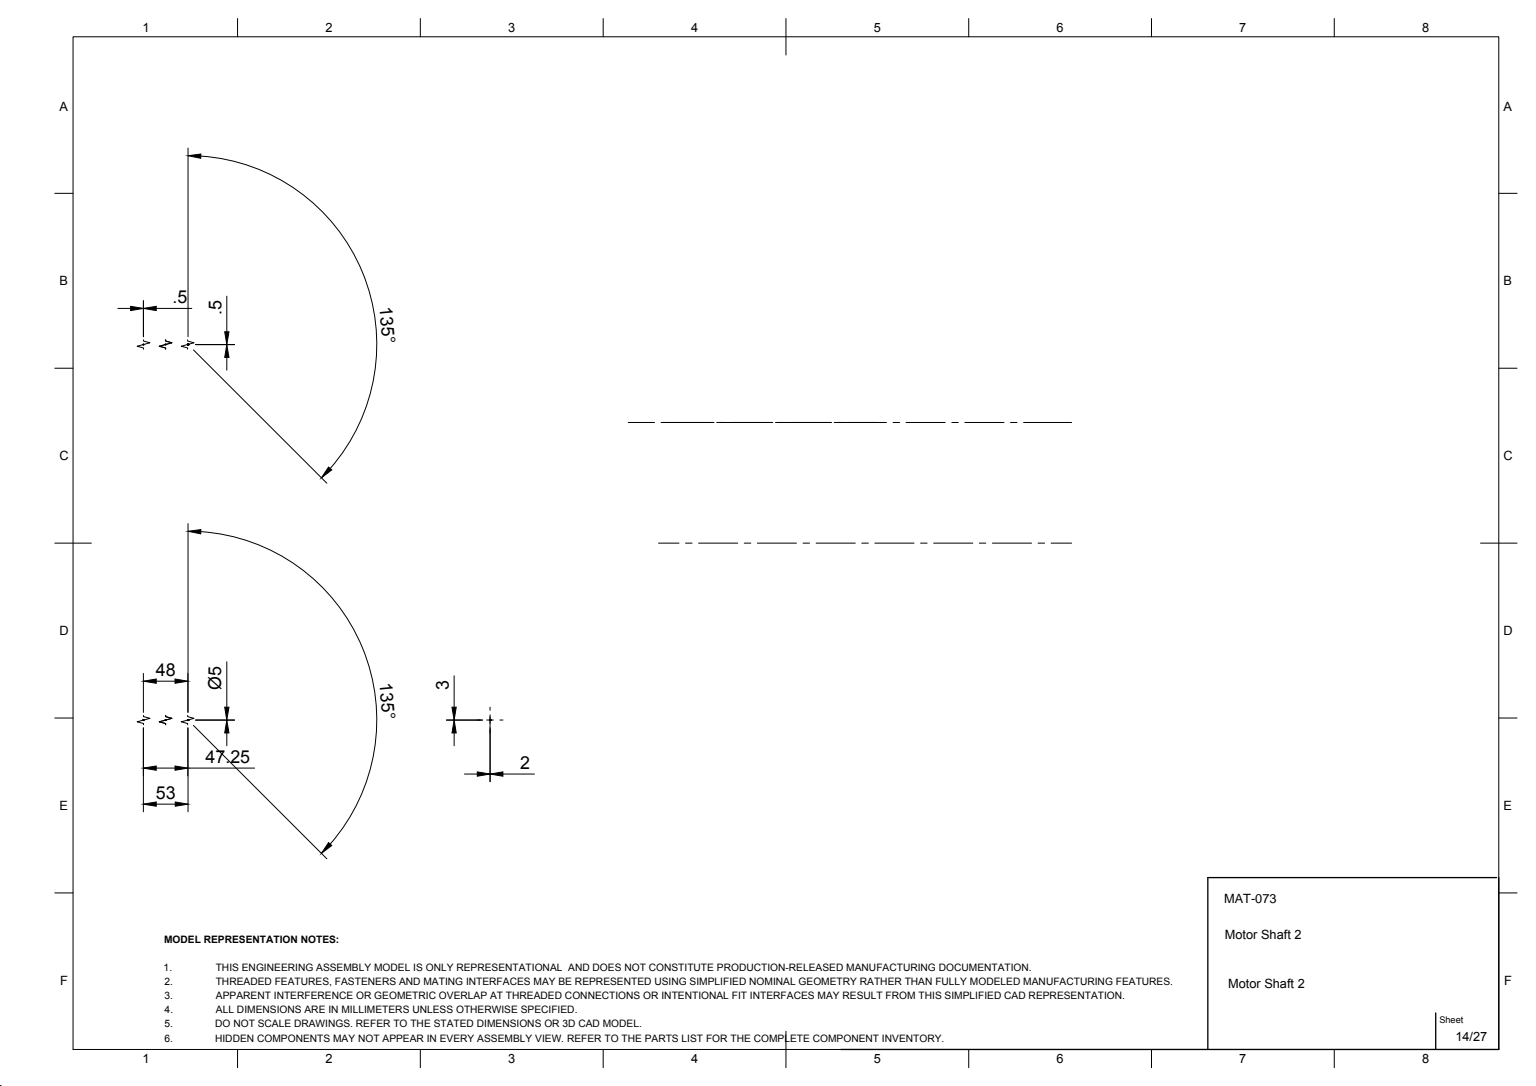
ISO-10303-21;
HEADER;
/* Generated by software containing ST-Developer
 * from STEP Tools, Inc. (www.steptools.com) 
 */

FILE_DESCRIPTION(
/* description */ ('CAx-IF Rec.Pracs.---Representation and Presentation of Product Manufa
cturing Information (PMI)---4.0---2014-10-13'),
/* implementation_level */ '2;1');

FILE_NAME(
/* name */ 'Motor Shaft 2.step',
/* time_stamp */ '2026-10-24T18:52:33-07:00',
/* author */ (''),
/* organization */ (''),
/* preprocessor_version */ 'ST-DEVELOPER v20.2',
/* originating_system */ 'Autodesk Translation Framework v15.17.0.0',
/* authorisation */ '');

FILE_SCHEMA (('AP242_MANAGED_MODEL_BASED_3D_ENGINEERING_MIM_LF { 1 0 10303 442 2 1 4 }'));
ENDSEC;

DATA;
#10=MECHANICAL_DESIGN_GEOMETRIC_PRESENTATION_REPRESENTATION('',(#427),#34876);
#156=(
BOUNDED_CURVE()
B_SPLINE_CURVE(2,(#31813,#31814,#31815),.UNSPECIFIED.,.F.,.F.)
B_SPLINE_CURVE_WITH_KNOTS((3,3),(0.,0.159611859165466),.UNSPECIFIED.)
CURVE()
GEOMETRIC_REPRESENTATION_ITEM()
RATIONAL_B_SPLINE_CURVE((1.,1.06066017177976,1.))
REPRESENTATION_ITEM('')
);
#157=(
BOUNDED_CURVE()
B_SPLINE_CURVE(2,(#31820,#31821,#31822),.UNSPECIFIED.,.F.,.F.)
B_SPLINE_CURVE_WITH_KNOTS((3,3),(0.159611859165466,0.319223718330933),
 .UNSPECIFIED.)
CURVE()
GEOMETRIC_REPRESENTATION_ITEM()
RATIONAL_B_SPLINE_CURVE((1.,1.06066017177976,1.))
REPRESENTATION_ITEM('')
);
#185=CONICAL_SURFACE('',#21171,0.00225,0.78539816339745);
#186=CONICAL_SURFACE('',#21175,0.00225,0.78539816339745);
#187=CONICAL_SURFACE('',#21192,0.00225,0.78539816339745);
#361=SHAPE_REPRESENTATION_RELATIONSHIP('SRR','None',#34998,#394);
#394=ADVANCED_BREP_SHAPE_REPRESENTATION('',(#460),#34856);
#427=STYLED_ITEM('',(#35159),#460);
#460=MANIFOLD_SOLID_BREP('Motor Shaft 2',#19567);
#534=FACE_BOUND('',#6448,.T.);
#535=FACE_BOUND('',#6450,.T.);
#861=PLANE('',#21181);
#862=PLANE('',#21183);
#863=PLANE('',#21187);
#864=PLANE('',#21188);
#865=PLANE('',#21194);
#866=PLANE('',#21195);
#1899=LINE('',#31807,#3498);
#1900=LINE('',#31828,#3499);
#1901=LINE('',#31838,#3500);
#1902=LINE('',#31839,#3501);
#1903=LINE('',#31841,#3502);
#1904=LINE('',#31844,#3503);
#1905=LINE('',#31848,#3504);
#1906=LINE('',#31854,#3505);
#3498=VECTOR('',#25516,0.00225);
#3499=VECTOR('',#25533,0.002);
#3500=VECTOR('',#25546,1.);
#3501=VECTOR('',#25547,0.0025);
#3502=VECTOR('',#25548,1.);
#3503=VECTOR('',#25553,1.);
#3504=VECTOR('',#25558,0.0025);
#3505=VECTOR('',#25565,0.00225);
#4547=CYLINDRICAL_SURFACE('',#21178,0.002);
#4548=CYLINDRICAL_SURFACE('',#21185,0.0025);
#4549=CYLINDRICAL_SURFACE('',#21189,0.0025);
#5345=FACE_OUTER_BOUND('',#6444,.T.);
#5346=FACE_OUTER_BOUND('',#6445,.T.);
#5347=FACE_OUTER_BOUND('',#6446,.T.);
#5348=FACE_OUTER_BOUND('',#6447,.T.);
#5349=FACE_OUTER_BOUND('',#6449,.T.);
#5350=FACE_OUTER_BOUND('',#6451,.T.);
#5351=FACE_OUTER_BOUND('',#6452,.T.);
#5352=FACE_OUTER_BOUND('',#6453,.T.);
#5353=FACE_OUTER_BOUND('',#6454,.T.);
#5354=FACE_OUTER_BOUND('',#6455,.T.);
#5355=FACE_OUTER_BOUND('',#6456,.T.);
#5356=FACE_OUTER_BOUND('',#6457,.T.);
#6444=EDGE_LOOP('',(#15784,#15785,#15786,#15787,#15788));
#6445=EDGE_LOOP('',(#15789,#15790,#15791,#15792));
#6446=EDGE_LOOP('',(#15793,#15794,#15795,#15796));
#6447=EDGE_LOOP('',(#15797));
#6448=EDGE_LOOP('',(#15798));
#6449=EDGE_LOOP('',(#15799));
#6450=EDGE_LOOP('',(#15800));
#6451=EDGE_LOOP('',(#15801,#15802,#15803,#15804,#15805,#15806,#15807,#15808,
#15809));
#6452=EDGE_LOOP('',(#15810,#15811,#15812,#15813,#15814));
#6453=EDGE_LOOP('',(#15815,#15816));
#6454=EDGE_LOOP('',(#15817,#15818,#15819,#15820,#15821));
#6455=EDGE_LOOP('',(#15822,#15823,#15824,#15825,#15826));
#6456=EDGE_LOOP('',(#15827));
#6457=EDGE_LOOP('',(#15828,#15829));
#7534=CIRCLE('',#21172,0.00250000000001);
#7535=CIRCLE('',#21173,0.00250000000001);
#7536=CIRCLE('',#21174,0.00200000000001);
#7537=CIRCLE('',#21176,0.00200000000001);
#7538=CIRCLE('',#21177,0.00250000000001);
#7539=CIRCLE('',#21179,0.00200000000001);
#7540=CIRCLE('',#21180,0.00200000000001);
#7541=CIRCLE('',#21182,0.00250000000001);
#7542=CIRCLE('',#21184,0.00250000000001);
#7543=CIRCLE('',#21186,0.00250000000001);
#7544=CIRCLE('',#21190,0.00250000000001);
#7545=CIRCLE('',#21191,0.00250000000001);
#7546=CIRCLE('',#21193,0.00200000000001);
#9058=VERTEX_POINT('',#31805);
#9059=VERTEX_POINT('',#31806);
#9060=VERTEX_POINT('',#31808);
#9061=VERTEX_POINT('',#31810);
#9062=VERTEX_POINT('',#31812);
#9063=VERTEX_POINT('',#31819);
#9064=VERTEX_POINT('',#31825);
#9065=VERTEX_POINT('',#31827);
#9066=VERTEX_POINT('',#31831);
#9067=VERTEX_POINT('',#31834);
#9068=VERTEX_POINT('',#31837);
#9069=VERTEX_POINT('',#31840);
#9070=VERTEX_POINT('',#31847);
#9071=VERTEX_POINT('',#31849);
#9072=VERTEX_POINT('',#31853);
#11450=EDGE_CURVE('',#9058,#9059,#1899,.T.);
#11451=EDGE_CURVE('',#9058,#9060,#7534,.T.);
#11452=EDGE_CURVE('',#9060,#9061,#7535,.T.);
#11453=EDGE_CURVE('',#9061,#9062,#156,.T.);
#11454=EDGE_CURVE('',#9062,#9059,#7536,.T.);
#11455=EDGE_CURVE('',#9059,#9062,#7537,.T.);
#11456=EDGE_CURVE('',#9062,#9063,#157,.T.);
#11457=EDGE_CURVE('',#9063,#9058,#7538,.T.);
#11458=EDGE_CURVE('',#9064,#9064,#7539,.T.);
#11459=EDGE_CURVE('',#9064,#9065,#1900,.T.);
#11460=EDGE_CURVE('',#9065,#9065,#7540,.T.);
#11461=EDGE_CURVE('',#9066,#9066,#7541,.T.);
#11462=EDGE_CURVE('',#9067,#9067,#7542,.T.);
#11463=EDGE_CURVE('',#9068,#9061,#1901,.T.);
#11464=EDGE_CURVE('',#9060,#9067,#1902,.T.);
#11465=EDGE_CURVE('',#9063,#9069,#1903,.T.);
#11466=EDGE_CURVE('',#9069,#9068,#7543,.T.);
#11467=EDGE_CURVE('',#9068,#9069,#1904,.T.);
#11468=EDGE_CURVE('',#9066,#9070,#1905,.T.);
#11469=EDGE_CURVE('',#9071,#9070,#7544,.T.);
#11470=EDGE_CURVE('',#9070,#9071,#7545,.T.);
#11471=EDGE_CURVE('',#9071,#9072,#1906,.T.);
#11472=EDGE_CURVE('',#9072,#9072,#7546,.T.);
#15784=ORIENTED_EDGE('',*,*,#11450,.F.);
#15785=ORIENTED_EDGE('',*,*,#11451,.T.);
#15786=ORIENTED_EDGE('',*,*,#11452,.T.);
#15787=ORIENTED_EDGE('',*,*,#11453,.T.);
#15788=ORIENTED_EDGE('',*,*,#11454,.T.);
#15789=ORIENTED_EDGE('',*,*,#11450,.T.);
#15790=ORIENTED_EDGE('',*,*,#11455,.T.);
#15791=ORIENTED_EDGE('',*,*,#11456,.T.);
#15792=ORIENTED_EDGE('',*,*,#11457,.T.);
#15793=ORIENTED_EDGE('',*,*,#11458,.T.);
#15794=ORIENTED_EDGE('',*,*,#11459,.T.);
#15795=ORIENTED_EDGE('',*,*,#11460,.T.);
#15796=ORIENTED_EDGE('',*,*,#11459,.F.);
#15797=ORIENTED_EDGE('',*,*,#11461,.F.);
#15798=ORIENTED_EDGE('',*,*,#11460,.F.);
#15799=ORIENTED_EDGE('',*,*,#11462,.F.);
#15800=ORIENTED_EDGE('',*,*,#11458,.F.);
#15801=ORIENTED_EDGE('',*,*,#11463,.T.);
#15802=ORIENTED_EDGE('',*,*,#11452,.F.);
#15803=ORIENTED_EDGE('',*,*,#11464,.T.);
#15804=ORIENTED_EDGE('',*,*,#11462,.T.);
#15805=ORIENTED_EDGE('',*,*,#11464,.F.);
#15806=ORIENTED_EDGE('',*,*,#11451,.F.);
#15807=ORIENTED_EDGE('',*,*,#11457,.F.);
#15808=ORIENTED_EDGE('',*,*,#11465,.T.);
#15809=ORIENTED_EDGE('',*,*,#11466,.T.);
#15810=ORIENTED_EDGE('',*,*,#11453,.F.);
#15811=ORIENTED_EDGE('',*,*,#11463,.F.);
#15812=ORIENTED_EDGE('',*,*,#11467,.T.);
#15813=ORIENTED_EDGE('',*,*,#11465,.F.);
#15814=ORIENTED_EDGE('',*,*,#11456,.F.);
#15815=ORIENTED_EDGE('',*,*,#11466,.F.);
#15816=ORIENTED_EDGE('',*,*,#11467,.F.);
#15817=ORIENTED_EDGE('',*,*,#11461,.T.);
#15818=ORIENTED_EDGE('',*,*,#11468,.T.);
#15819=ORIENTED_EDGE('',*,*,#11469,.F.);
#15820=ORIENTED_EDGE('',*,*,#11470,.F.);
#15821=ORIENTED_EDGE('',*,*,#11468,.F.);
#15822=ORIENTED_EDGE('',*,*,#11470,.T.);
#15823=ORIENTED_EDGE('',*,*,#11471,.T.);
#15824=ORIENTED_EDGE('',*,*,#11472,.T.);
#15825=ORIENTED_EDGE('',*,*,#11471,.F.);
#15826=ORIENTED_EDGE('',*,*,#11469,.T.);
#15827=ORIENTED_EDGE('',*,*,#11472,.F.);
#15828=ORIENTED_EDGE('',*,*,#11454,.F.);
#15829=ORIENTED_EDGE('',*,*,#11455,.F.);
#19061=ADVANCED_FACE('',(#5345),#185,.T.);
#19062=ADVANCED_FACE('',(#5346),#186,.T.);
#19063=ADVANCED_FACE('',(#5347),#4547,.T.);
#19064=ADVANCED_FACE('',(#5348,#534),#861,.F.);
#19065=ADVANCED_FACE('',(#5349,#535),#862,.T.);
#19066=ADVANCED_FACE('',(#5350),#4548,.T.);
#19067=ADVANCED_FACE('',(#5351),#863,.F.);
#19068=ADVANCED_FACE('',(#5352),#864,.F.);
#19069=ADVANCED_FACE('',(#5353),#4549,.T.);
#19070=ADVANCED_FACE('',(#5354),#187,.T.);
#19071=ADVANCED_FACE('',(#5355),#865,.F.);
#19072=ADVANCED_FACE('',(#5356),#866,.T.);
#19567=CLOSED_SHELL('',(#19061,#19062,#19063,#19064,#19065,#19066,#19067,
#19068,#19069,#19070,#19071,#19072));
#21170=AXIS2_PLACEMENT_3D('',#31803,#25512,#25513);
#21171=AXIS2_PLACEMENT_3D('',#31804,#25514,#25515);
#21172=AXIS2_PLACEMENT_3D('',#31809,#25517,#25518);
#21173=AXIS2_PLACEMENT_3D('',#31811,#25519,#25520);
#21174=AXIS2_PLACEMENT_3D('',#31816,#25521,#25522);
#21175=AXIS2_PLACEMENT_3D('',#31817,#25523,#25524);
#21176=AXIS2_PLACEMENT_3D('',#31818,#25525,#25526);
#21177=AXIS2_PLACEMENT_3D('',#31823,#25527,#25528);
#21178=AXIS2_PLACEMENT_3D('',#31824,#25529,#25530);
#21179=AXIS2_PLACEMENT_3D('',#31826,#25531,#25532);
#21180=AXIS2_PLACEMENT_3D('',#31829,#25534,#25535);
#21181=AXIS2_PLACEMENT_3D('',#31830,#25536,#25537);
#21182=AXIS2_PLACEMENT_3D('',#31832,#25538,#25539);
#21183=AXIS2_PLACEMENT_3D('',#31833,#25540,#25541);
#21184=AXIS2_PLACEMENT_3D('',#31835,#25542,#25543);
#21185=AXIS2_PLACEMENT_3D('',#31836,#25544,#25545);
#21186=AXIS2_PLACEMENT_3D('',#31842,#25549,#25550);
#21187=AXIS2_PLACEMENT_3D('',#31843,#25551,#25552);
#21188=AXIS2_PLACEMENT_3D('',#31845,#25554,#25555);
#21189=AXIS2_PLACEMENT_3D('',#31846,#25556,#25557);
#21190=AXIS2_PLACEMENT_3D('',#31850,#25559,#25560);
#21191=AXIS2_PLACEMENT_3D('',#31851,#25561,#25562);
#21192=AXIS2_PLACEMENT_3D('',#31852,#25563,#25564);
#21193=AXIS2_PLACEMENT_3D('',#31855,#25566,#25567);
#21194=AXIS2_PLACEMENT_3D('',#31856,#25568,#25569);
#21195=AXIS2_PLACEMENT_3D('',#31857,#25570,#25571);
#25512=DIRECTION('axis',(0.,0.,1.));
#25513=DIRECTION('refdir',(1.,0.,0.));
#25514=DIRECTION('center_axis',(6.65798752924967E-17,-1.,1.71022579061586E-31));
#25515=DIRECTION('ref_axis',(-0.211873077029416,-1.41064830464559E-17,0.97729719084324));
#25516=DIRECTION('',(-0.14981688951836,0.707106781186546,0.691053470879819));
#25517=DIRECTION('center_axis',(-6.65798752924967E-17,1.,-1.71022579061586E-31));
#25518=DIRECTION('ref_axis',(-0.211873077029416,-1.41064830464559E-17,0.977297190843239));
#25519=DIRECTION('center_axis',(-6.65798752924967E-17,1.,-1.71022579061586E-31));
#25520=DIRECTION('ref_axis',(-0.211873077029416,-1.41064830464559E-17,0.977297190843239));
#25521=DIRECTION('center_axis',(6.65798752924967E-17,-1.,1.71022579061586E-31));
#25522=DIRECTION('ref_axis',(-0.211873077029416,-1.41064830464559E-17,0.97729719084324));
#25523=DIRECTION('center_axis',(6.65798752924967E-17,-1.,1.71022579061586E-31));
#25524=DIRECTION('ref_axis',(-0.211873077029416,-1.41064830464559E-17,0.97729719084324));
#25525=DIRECTION('center_axis',(6.65798752924967E-17,-1.,1.71022579061586E-31));
#25526=DIRECTION('ref_axis',(-0.211873077029416,-1.41064830464559E-17,0.97729719084324));
#25527=DIRECTION('center_axis',(-6.65798752924967E-17,1.,-1.71022579061586E-31));
#25528=DIRECTION('ref_axis',(-0.211873077029416,-1.41064830464559E-17,0.977297190843239));
#25529=DIRECTION('center_axis',(-6.65798752924967E-17,1.,-1.71022579061586E-31));
#25530=DIRECTION('ref_axis',(0.211873077029416,1.41064830464559E-17,-0.977297190843239));
#25531=DIRECTION('center_axis',(6.65798752924967E-17,-1.,1.71022579061586E-31));
#25532=DIRECTION('ref_axis',(0.211873077029416,1.41064830464559E-17,-0.97729719084324));
#25533=DIRECTION('',(6.65798752924967E-17,-1.,1.71022579061586E-31));
#25534=DIRECTION('center_axis',(-6.65798752924967E-17,1.,-1.71022579061586E-31));
#25535=DIRECTION('ref_axis',(0.211873077029416,1.41064830464559E-17,-0.97729719084324));
#25536=DIRECTION('center_axis',(6.65798752924967E-17,-1.,1.71022579061586E-31));
#25537=DIRECTION('ref_axis',(0.97729719084324,6.50683250900503E-17,0.211873077029416));
#25538=DIRECTION('center_axis',(6.65798752924967E-17,-1.,1.71022579061586E-31));
#25539=DIRECTION('ref_axis',(0.211873077029416,1.41064830464559E-17,-0.977297190843239));
#25540=DIRECTION('center_axis',(6.65798752924967E-17,-1.,1.71022579061586E-31));
#25541=DIRECTION('ref_axis',(0.97729719084324,6.50683250900503E-17,0.211873077029416));
#25542=DIRECTION('center_axis',(-6.65798752924967E-17,1.,-1.71022579061586E-31));
#25543=DIRECTION('ref_axis',(0.211873077029416,1.41064830464559E-17,-0.977297190843239));
#25544=DIRECTION('center_axis',(-6.65798752924967E-17,1.,-1.71022579061586E-31));
#25545=DIRECTION('ref_axis',(0.211873077029416,1.41064830464559E-17,-0.97729719084324));
#25546=DIRECTION('',(-6.65798752924967E-17,1.,-1.71022579061586E-31));
#25547=DIRECTION('',(6.65798752924967E-17,-1.,1.71022579061586E-31));
#25548=DIRECTION('',(6.65798752924967E-17,-1.,1.71022579061586E-31));
#25549=DIRECTION('center_axis',(6.65798752924967E-17,-1.,1.71022579061586E-31));
#25550=DIRECTION('ref_axis',(0.211873077029416,1.41064830464559E-17,-0.977297190843239));
#25551=DIRECTION('center_axis',(-0.97729719084324,-6.50683250900503E-17,
-0.211873077029416));
#25552=DIRECTION('ref_axis',(-0.211873077029416,-1.06625068431886E-16,0.97729719084324));
#25553=DIRECTION('',(0.211873077028438,1.41064830463908E-17,-0.977297190843451));
#25554=DIRECTION('center_axis',(6.65798752924967E-17,-1.,1.71022579061586E-31));
#25555=DIRECTION('ref_axis',(0.97729719084324,6.50683250900503E-17,0.211873077029416));
#25556=DIRECTION('center_axis',(-6.65798752924967E-17,1.,-1.71022579061586E-31));
#25557=DIRECTION('ref_axis',(0.211873077029416,1.41064830464559E-17,-0.97729719084324));
#25558=DIRECTION('',(6.65798752924967E-17,-1.,1.71022579061586E-31));
#25559=DIRECTION('center_axis',(6.65798752924967E-17,-1.,1.71022579061586E-31));
#25560=DIRECTION('ref_axis',(-0.211873077029416,-1.41064830464559E-17,0.977297190843239));
#25561=DIRECTION('center_axis',(6.65798752924967E-17,-1.,1.71022579061586E-31));
#25562=DIRECTION('ref_axis',(-0.211873077029416,-1.41064830464559E-17,0.977297190843239));
#25563=DIRECTION('center_axis',(-6.65798752924967E-17,1.,-1.71022579061586E-31));
#25564=DIRECTION('ref_axis',(-0.211873077029416,-1.41064830464559E-17,0.97729719084324));
#25565=DIRECTION('',(-0.14981688951836,-0.707106781186546,0.691053470879819));
#25566=DIRECTION('center_axis',(-6.65798752924967E-17,1.,-1.71022579061586E-31));
#25567=DIRECTION('ref_axis',(-0.211873077029416,-1.41064830464559E-17,0.97729719084324));
#25568=DIRECTION('center_axis',(-6.65798752924967E-17,1.,-1.71022579061586E-31));
#25569=DIRECTION('ref_axis',(-0.211873077029416,-1.41064830464559E-17,0.97729719084324));
#25570=DIRECTION('center_axis',(-6.65798752924967E-17,1.,-1.71022579061586E-31));
#25571=DIRECTION('ref_axis',(-0.211873077029416,-1.41064830464559E-17,0.97729719084324));
#31803=CARTESIAN_POINT('',(0.,0.,0.));
#31804=CARTESIAN_POINT('Origin',(-4.68201057504096E-17,0.0215,5.80537005579265E-33));
#31805=CARTESIAN_POINT('',(0.000529682692573917,0.021249999999998,-0.00244324297711006));
#31806=CARTESIAN_POINT('',(0.000423746154058535,0.0217500000000012,-0.00195459438168533));
#31807=CARTESIAN_POINT('',(0.000476714423316139,0.0215,-0.00219891867939729));
#31808=CARTESIAN_POINT('',(-0.000529682692573586,0.02125000000001,0.0024432429771081));
#31809=CARTESIAN_POINT('Origin',(-4.68034607815872E-17,0.02125000000001,
5.84812570055634E-33));
#31810=CARTESIAN_POINT('',(0.00163678476614231,0.02125,0.00188969194032369));
#31811=CARTESIAN_POINT('Origin',(-4.68034607815872E-17,0.02125000000001,
5.84812570055634E-33));
#31812=CARTESIAN_POINT('',(0.00195459438168643,0.02175,0.000423746154058832));
#31813=CARTESIAN_POINT('Ctrl Pts',(0.00163678476614996,0.02125000000001,
0.00188969194033559));
#31814=CARTESIAN_POINT('Ctrl Pts',(0.00181334566367447,0.02175000000001,
0.0010752776146329));
#31815=CARTESIAN_POINT('Ctrl Pts',(0.00195459438169832,0.02175000000001,
0.000423746154051177));
#31816=CARTESIAN_POINT('Origin',(-4.68367507192334E-17,0.02175000000001,
5.76261441102555E-33));
#31817=CARTESIAN_POINT('Origin',(-4.68201057504096E-17,0.0215,5.80537005579265E-33));
#31818=CARTESIAN_POINT('Origin',(-4.68367507192334E-17,0.02175000000001,
5.76261441102555E-33));
#31819=CARTESIAN_POINT('',(0.00227240399723056,0.02125,-0.00104219963220603));
#31820=CARTESIAN_POINT('Ctrl Pts',(0.00195459438169832,0.02175000000001,
0.000423746154051177));
#31821=CARTESIAN_POINT('Ctrl Pts',(0.00209584309971794,0.02175000000001,
-0.000227785306511001));
#31822=CARTESIAN_POINT('Ctrl Pts',(0.00227240399724245,0.02125000000001,
-0.00104219963221369));
#31823=CARTESIAN_POINT('Origin',(-4.68034607815872E-17,0.02125000000001,
5.84812570055634E-33));
#31824=CARTESIAN_POINT('Origin',(-4.36409167051929E-17,-0.02625,1.39716982059834E-32));
#31825=CARTESIAN_POINT('',(-0.000423746154058875,-0.02550000000001,0.00195459438168648));
#31826=CARTESIAN_POINT('Origin',(-4.36908516116616E-17,-0.02550000000001,
1.38434312716889E-32));
#31827=CARTESIAN_POINT('',(-0.000423746154058875,-0.02625000000001,0.00195459438168648));
#31828=CARTESIAN_POINT('',(-0.000423746154058875,-0.02625,0.00195459438168648));
#31829=CARTESIAN_POINT('Origin',(-4.36409167051922E-17,-0.02625000000001,
1.39716982059851E-32));
#31830=CARTESIAN_POINT('Origin',(-4.36409167051929E-17,-0.02625,1.39716982059834E-32));
#31831=CARTESIAN_POINT('',(-0.000529682692573583,-0.02625000000001,0.0024432429771081));
#31832=CARTESIAN_POINT('Origin',(-4.36409167051922E-17,-0.02625000000001,
1.39716982059851E-32));
#31833=CARTESIAN_POINT('Origin',(-4.36908516116622E-17,-0.0255,1.38434312716872E-32));
#31834=CARTESIAN_POINT('',(-0.000529682692573583,-0.02550000000001,0.0024432429771081));
#31835=CARTESIAN_POINT('Origin',(-4.36908516116616E-17,-0.02550000000001,
1.38434312716889E-32));
#31836=CARTESIAN_POINT('Origin',(-4.50723840239816E-17,-0.00475,1.02947127561593E-32));
#31837=CARTESIAN_POINT('',(0.00163678476614231,0.00375,0.00188969194032369));
#31838=CARTESIAN_POINT('',(0.00163678476614996,-0.00475,0.00188969194033558));
#31839=CARTESIAN_POINT('',(-0.000529682692573585,-0.00475,0.0024432429771081));
#31840=CARTESIAN_POINT('',(0.00227240399723056,0.00375,-0.00104219963220603));
#31841=CARTESIAN_POINT('',(0.00227240399724245,-0.00475,-0.00104219963221368));
#31842=CARTESIAN_POINT('Origin',(-4.56383129639685E-17,0.00375000000001,
8.8410208341341E-33));
#31843=CARTESIAN_POINT('Origin',(0.00163678476614231,0.02175,0.00188969194032369));
#31844=CARTESIAN_POINT('',(0.00227240399724245,0.00375000000001,-0.00104219963221368));
#31845=CARTESIAN_POINT('Origin',(0.00219891867939725,0.00375,0.000476714423316185));
#31846=CARTESIAN_POINT('Origin',(-4.50723840239816E-17,-0.00475,1.02947127561593E-32));
#31847=CARTESIAN_POINT('',(-0.000529682692575702,-0.03075000000001,0.00244324297711787));
#31848=CARTESIAN_POINT('',(-0.000529682692573585,-0.00475,0.0024432429771081));
#31849=CARTESIAN_POINT('',(0.000529682692573497,-0.03075,-0.0024432429771081));
#31850=CARTESIAN_POINT('Origin',(-4.3341307266376E-17,-0.03075000000001,
1.47412998117623E-32));
#31851=CARTESIAN_POINT('Origin',(-4.3341307266376E-17,-0.03075000000001,
1.47412998117623E-32));
#31852=CARTESIAN_POINT('Origin',(-4.33246622975535E-17,-0.031,1.47840554565259E-32));
#31853=CARTESIAN_POINT('',(0.000423746154058788,-0.03125,-0.00195459438168648));
#31854=CARTESIAN_POINT('',(0.000476714423316142,-0.031,-0.00219891867939729));
#31855=CARTESIAN_POINT('Origin',(-4.33080173287297E-17,-0.03125000000001,
1.4826811101293E-32));
#31856=CARTESIAN_POINT('Origin',(-4.33080173287304E-17,-0.03125,1.48268111012913E-32));
#31857=CARTESIAN_POINT('Origin',(-4.68367507192327E-17,0.02175,5.76261441102726E-33));
#34821=UNCERTAINTY_MEASURE_WITH_UNIT(LENGTH_MEASURE(1.E-5),#34877,
'DISTANCE_ACCURACY_VALUE',
'Maximum model space distance between geometric entities at asserted c
onnectivities');
#34841=UNCERTAINTY_MEASURE_WITH_UNIT(LENGTH_MEASURE(1.E-5),#34877,
'DISTANCE_ACCURACY_VALUE',
'Maximum model space distance between geometric entities at asserted c
onnectivities');
#34856=(
GEOMETRIC_REPRESENTATION_CONTEXT(3)
GLOBAL_UNCERTAINTY_ASSIGNED_CONTEXT((#34821))
GLOBAL_UNIT_ASSIGNED_CONTEXT((#34877,#34878,#34879))
REPRESENTATION_CONTEXT('','3D')
);
#34876=(
GEOMETRIC_REPRESENTATION_CONTEXT(3)
GLOBAL_UNCERTAINTY_ASSIGNED_CONTEXT((#34841))
GLOBAL_UNIT_ASSIGNED_CONTEXT((#34877,#34878,#34879))
REPRESENTATION_CONTEXT('','3D')
);
#34877=(
LENGTH_UNIT()
NAMED_UNIT(*)
SI_UNIT($,.METRE.)
);
#34878=(
NAMED_UNIT(*)
PLANE_ANGLE_UNIT()
SI_UNIT($,.RADIAN.)
);
#34879=(
NAMED_UNIT(*)
SI_UNIT($,.STERADIAN.)
SOLID_ANGLE_UNIT()
);
#34894=SHAPE_DEFINITION_REPRESENTATION(#34928,#34998);
#34928=PRODUCT_DEFINITION_SHAPE('',$,#35033);
#34998=SHAPE_REPRESENTATION('',(#21170),#34856);
#35018=PRODUCT_DEFINITION_CONTEXT('part definition',#35122,'design');
#35033=PRODUCT_DEFINITION('Motor Shaft 2','Motor Shaft 2',#35067,#35018);
#35067=PRODUCT_DEFINITION_FORMATION('',$,#35138);
#35122=APPLICATION_CONTEXT('Managed model based 3d engineering');
#35123=PRODUCT_CONTEXT('part definition',#35122,'mechanical');
#35138=PRODUCT('Motor Shaft 2','Motor Shaft 2',
'LEGAL AND USAGE DISCLAIMER: this Data/Model is provided \X2\201C\X0\A
S IS\X2\201D\X0\ for informational and representational only. It is a 
geometric approximation and is NOT engineered, certified, or guarantee
d for dimensional accuracy, exact tolerances, or production-level prec
ision. Vendor disclaims all implied warranties including fitness for a
 particular purpose. DO NOT USE FOR DIRECT PHYSICAL MANUFACTURING, AUT
OMATED PRODUCTION, OR SAFETY-CRITICAL SYSTEMS without independent engi
neering verification and resolution of any design discrepancies.',(#35123));
#35159=PRESENTATION_STYLE_ASSIGNMENT((#35168));
#35168=SURFACE_STYLE_USAGE(.BOTH.,#35177);
#35177=SURFACE_SIDE_STYLE('',(#35186));
#35186=SURFACE_STYLE_FILL_AREA(#35195);
#35195=FILL_AREA_STYLE('Paint - Enamel Glossy (White)',(#35204));
#35204=FILL_AREA_STYLE_COLOUR('Paint - Enamel Glossy (White)',#35213);
#35213=COLOUR_RGB('Paint - Enamel Glossy (White)',0.964705882352941,0.964705882352941,
0.952941176470588);
ENDSEC;
END-ISO-10303-21;
